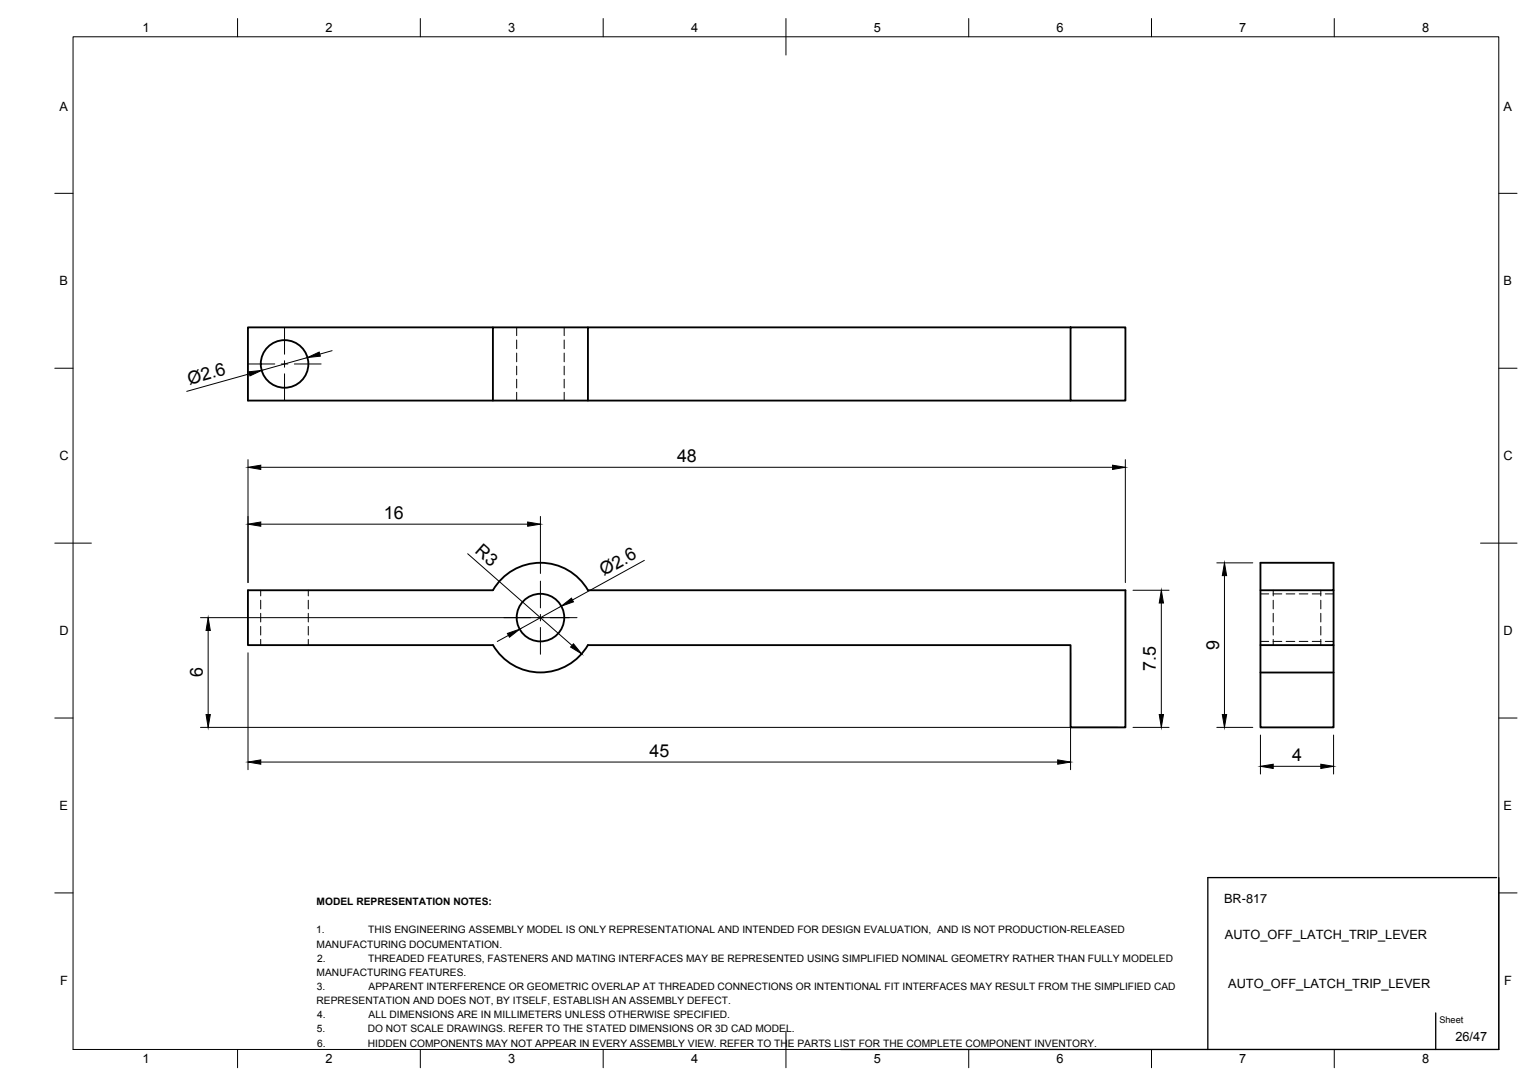
ISO-10303-21;
HEADER;
FILE_DESCRIPTION((''),'2;1');
FILE_NAME('AUTO_OFF_LATCH_TRIP_LEVER.step','2026-10-01T22:07:29-07:00',(''),(''),'','','');
FILE_SCHEMA (('AUTOMOTIVE_DESIGN { 1 0 10303 214 3 1 1 }'));
ENDSEC;
DATA;
#10=MECHANICAL_DESIGN_GEOMETRIC_PRESENTATION_REPRESENTATION('',(#558),#15484);
#488=SHAPE_REPRESENTATION_RELATIONSHIP('SRR','None',#15638,#523) ;
#523=ADVANCED_BREP_SHAPE_REPRESENTATION('',(#599),#15462) ;
#558=STYLED_ITEM('',(#15833),#599) ;
#599=MANIFOLD_SOLID_BREP('AUTO_OFF_LATCH_TRIP_LEVER',#8269) ;
#682=CYLINDRICAL_SURFACE('',#9012,0.13) ;
#683=CYLINDRICAL_SURFACE('',#9023,0.13) ;
#684=CYLINDRICAL_SURFACE('',#9025,0.3) ;
#685=CYLINDRICAL_SURFACE('',#9027,0.3) ;
#866=FACE_BOUND('',#2096,.T.) ;
#867=FACE_BOUND('',#2102,.T.) ;
#868=FACE_BOUND('',#2105,.T.) ;
#869=FACE_BOUND('',#2107,.T.) ;
#1007=CIRCLE('',#9013,0.13) ;
#1008=CIRCLE('',#9014,0.13) ;
#1009=CIRCLE('',#9019,0.3) ;
#1010=CIRCLE('',#9020,0.3) ;
#1011=CIRCLE('',#9021,0.13) ;
#1012=CIRCLE('',#9024,0.13) ;
#1013=CIRCLE('',#9026,0.3) ;
#1014=CIRCLE('',#9028,0.3) ;
#1535=FACE_OUTER_BOUND('',#2091,.T.) ;
#1536=FACE_OUTER_BOUND('',#2092,.T.) ;
#1537=FACE_OUTER_BOUND('',#2093,.T.) ;
#1538=FACE_OUTER_BOUND('',#2094,.T.) ;
#1539=FACE_OUTER_BOUND('',#2095,.T.) ;
#1540=FACE_OUTER_BOUND('',#2097,.T.) ;
#1541=FACE_OUTER_BOUND('',#2098,.T.) ;
#1542=FACE_OUTER_BOUND('',#2099,.T.) ;
#1543=FACE_OUTER_BOUND('',#2100,.T.) ;
#1544=FACE_OUTER_BOUND('',#2101,.T.) ;
#1545=FACE_OUTER_BOUND('',#2103,.T.) ;
#1546=FACE_OUTER_BOUND('',#2104,.T.) ;
#1547=FACE_OUTER_BOUND('',#2106,.T.) ;
#1548=FACE_OUTER_BOUND('',#2108,.T.) ;
#2091=EDGE_LOOP('',(#5943,#5944,#5945,#5946)) ;
#2092=EDGE_LOOP('',(#5947,#5948,#5949,#5950)) ;
#2093=EDGE_LOOP('',(#5951,#5952,#5953,#5954)) ;
#2094=EDGE_LOOP('',(#5955,#5956,#5957,#5958)) ;
#2095=EDGE_LOOP('',(#5959,#5960,#5961,#5962,#5963,#5964,#5965,#5966,#5967,
#5968)) ;
#2096=EDGE_LOOP('',(#5969)) ;
#2097=EDGE_LOOP('',(#5970,#5971,#5972,#5973)) ;
#2098=EDGE_LOOP('',(#5974,#5975,#5976,#5977)) ;
#2099=EDGE_LOOP('',(#5978,#5979,#5980,#5981)) ;
#2100=EDGE_LOOP('',(#5982,#5983,#5984,#5985)) ;
#2101=EDGE_LOOP('',(#5986,#5987,#5988,#5989)) ;
#2102=EDGE_LOOP('',(#5990)) ;
#2103=EDGE_LOOP('',(#5991,#5992,#5993,#5994)) ;
#2104=EDGE_LOOP('',(#5995,#5996,#5997,#5998,#5999,#6000,#6001,#6002,#6003,
#6004)) ;
#2105=EDGE_LOOP('',(#6005)) ;
#2106=EDGE_LOOP('',(#6006,#6007,#6008,#6009)) ;
#2107=EDGE_LOOP('',(#6010)) ;
#2108=EDGE_LOOP('',(#6011,#6012,#6013,#6014)) ;
#2649=LINE('',#13697,#3123) ;
#2650=LINE('',#13702,#3124) ;
#2651=LINE('',#13704,#3125) ;
#2652=LINE('',#13706,#3126) ;
#2653=LINE('',#13707,#3127) ;
#2654=LINE('',#13710,#3128) ;
#2655=LINE('',#13712,#3129) ;
#2656=LINE('',#13713,#3130) ;
#2657=LINE('',#13717,#3131) ;
#2658=LINE('',#13718,#3132) ;
#2659=LINE('',#13719,#3133) ;
#2660=LINE('',#13722,#3134) ;
#2661=LINE('',#13726,#3135) ;
#2662=LINE('',#13728,#3136) ;
#2663=LINE('',#13730,#3137) ;
#2664=LINE('',#13733,#3138) ;
#2665=LINE('',#13738,#3139) ;
#2666=LINE('',#13739,#3140) ;
#2667=LINE('',#13742,#3141) ;
#2668=LINE('',#13747,#3142) ;
#2669=LINE('',#13750,#3143) ;
#2670=LINE('',#13752,#3144) ;
#2671=LINE('',#13756,#3145) ;
#2672=LINE('',#13757,#3146) ;
#2673=LINE('',#13759,#3147) ;
#2674=LINE('',#13762,#3148) ;
#2675=LINE('',#13763,#3149) ;
#2676=LINE('',#13765,#3150) ;
#3123=VECTOR('',#10798,0.13) ;
#3124=VECTOR('',#10803,1.) ;
#3125=VECTOR('',#10804,1.) ;
#3126=VECTOR('',#10805,1.) ;
#3127=VECTOR('',#10806,1.) ;
#3128=VECTOR('',#10809,1.) ;
#3129=VECTOR('',#10810,1.) ;
#3130=VECTOR('',#10811,1.) ;
#3131=VECTOR('',#10814,1.) ;
#3132=VECTOR('',#10815,1.) ;
#3133=VECTOR('',#10816,1.) ;
#3134=VECTOR('',#10819,1.) ;
#3135=VECTOR('',#10822,1.) ;
#3136=VECTOR('',#10823,1.) ;
#3137=VECTOR('',#10824,1.) ;
#3138=VECTOR('',#10827,1.) ;
#3139=VECTOR('',#10832,1.) ;
#3140=VECTOR('',#10833,1.) ;
#3141=VECTOR('',#10836,0.13) ;
#3142=VECTOR('',#10843,1.) ;
#3143=VECTOR('',#10846,1.) ;
#3144=VECTOR('',#10847,1.) ;
#3145=VECTOR('',#10852,1.) ;
#3146=VECTOR('',#10853,1.) ;
#3147=VECTOR('',#10856,1.) ;
#3148=VECTOR('',#10859,1.) ;
#3149=VECTOR('',#10860,1.) ;
#3150=VECTOR('',#10863,1.) ;
#3613=VERTEX_POINT('',#13694) ;
#3614=VERTEX_POINT('',#13696) ;
#3615=VERTEX_POINT('',#13700) ;
#3616=VERTEX_POINT('',#13701) ;
#3617=VERTEX_POINT('',#13703) ;
#3618=VERTEX_POINT('',#13705) ;
#3619=VERTEX_POINT('',#13709) ;
#3620=VERTEX_POINT('',#13711) ;
#3621=VERTEX_POINT('',#13715) ;
#3622=VERTEX_POINT('',#13716) ;
#3623=VERTEX_POINT('',#13721) ;
#3624=VERTEX_POINT('',#13723) ;
#3625=VERTEX_POINT('',#13725) ;
#3626=VERTEX_POINT('',#13727) ;
#3627=VERTEX_POINT('',#13729) ;
#3628=VERTEX_POINT('',#13731) ;
#3629=VERTEX_POINT('',#13734) ;
#3630=VERTEX_POINT('',#13737) ;
#3631=VERTEX_POINT('',#13741) ;
#3632=VERTEX_POINT('',#13745) ;
#3633=VERTEX_POINT('',#13749) ;
#3634=VERTEX_POINT('',#13751) ;
#3635=VERTEX_POINT('',#13755) ;
#3636=VERTEX_POINT('',#13761) ;
#4476=EDGE_CURVE('',#3613,#3613,#1007,.T.) ;
#4477=EDGE_CURVE('',#3613,#3614,#2649,.T.) ;
#4478=EDGE_CURVE('',#3614,#3614,#1008,.T.) ;
#4479=EDGE_CURVE('',#3615,#3616,#2650,.T.) ;
#4480=EDGE_CURVE('',#3616,#3617,#2651,.T.) ;
#4481=EDGE_CURVE('',#3617,#3618,#2652,.T.) ;
#4482=EDGE_CURVE('',#3618,#3615,#2653,.T.) ;
#4483=EDGE_CURVE('',#3619,#3618,#2654,.T.) ;
#4484=EDGE_CURVE('',#3620,#3617,#2655,.T.) ;
#4485=EDGE_CURVE('',#3619,#3620,#2656,.T.) ;
#4486=EDGE_CURVE('',#3621,#3622,#2657,.T.) ;
#4487=EDGE_CURVE('',#3621,#3616,#2658,.T.) ;
#4488=EDGE_CURVE('',#3622,#3615,#2659,.T.) ;
#4489=EDGE_CURVE('',#3623,#3621,#2660,.T.) ;
#4490=EDGE_CURVE('',#3623,#3624,#1009,.T.) ;
#4491=EDGE_CURVE('',#3625,#3624,#2661,.T.) ;
#4492=EDGE_CURVE('',#3626,#3625,#2662,.T.) ;
#4493=EDGE_CURVE('',#3627,#3626,#2663,.T.) ;
#4494=EDGE_CURVE('',#3627,#3628,#1010,.T.) ;
#4495=EDGE_CURVE('',#3620,#3628,#2664,.T.) ;
#4496=EDGE_CURVE('',#3629,#3629,#1011,.T.) ;
#4497=EDGE_CURVE('',#3622,#3630,#2665,.T.) ;
#4498=EDGE_CURVE('',#3630,#3623,#2666,.T.) ;
#4499=EDGE_CURVE('',#3629,#3631,#2667,.T.) ;
#4500=EDGE_CURVE('',#3631,#3631,#1012,.T.) ;
#4501=EDGE_CURVE('',#3632,#3630,#1013,.T.) ;
#4502=EDGE_CURVE('',#3624,#3632,#2668,.T.) ;
#4503=EDGE_CURVE('',#3628,#3633,#2669,.T.) ;
#4504=EDGE_CURVE('',#3634,#3627,#2670,.T.) ;
#4505=EDGE_CURVE('',#3633,#3634,#1014,.T.) ;
#4506=EDGE_CURVE('',#3626,#3635,#2671,.T.) ;
#4507=EDGE_CURVE('',#3635,#3634,#2672,.T.) ;
#4508=EDGE_CURVE('',#3633,#3619,#2673,.T.) ;
#4509=EDGE_CURVE('',#3635,#3636,#2674,.T.) ;
#4510=EDGE_CURVE('',#3632,#3636,#2675,.T.) ;
#4511=EDGE_CURVE('',#3636,#3625,#2676,.T.) ;
#5943=ORIENTED_EDGE('',*,*,#4476,.F.) ;
#5944=ORIENTED_EDGE('',*,*,#4477,.T.) ;
#5945=ORIENTED_EDGE('',*,*,#4478,.F.) ;
#5946=ORIENTED_EDGE('',*,*,#4477,.F.) ;
#5947=ORIENTED_EDGE('',*,*,#4479,.T.) ;
#5948=ORIENTED_EDGE('',*,*,#4480,.T.) ;
#5949=ORIENTED_EDGE('',*,*,#4481,.T.) ;
#5950=ORIENTED_EDGE('',*,*,#4482,.T.) ;
#5951=ORIENTED_EDGE('',*,*,#4483,.T.) ;
#5952=ORIENTED_EDGE('',*,*,#4481,.F.) ;
#5953=ORIENTED_EDGE('',*,*,#4484,.F.) ;
#5954=ORIENTED_EDGE('',*,*,#4485,.F.) ;
#5955=ORIENTED_EDGE('',*,*,#4486,.F.) ;
#5956=ORIENTED_EDGE('',*,*,#4487,.T.) ;
#5957=ORIENTED_EDGE('',*,*,#4479,.F.) ;
#5958=ORIENTED_EDGE('',*,*,#4488,.F.) ;
#5959=ORIENTED_EDGE('',*,*,#4489,.F.) ;
#5960=ORIENTED_EDGE('',*,*,#4490,.T.) ;
#5961=ORIENTED_EDGE('',*,*,#4491,.F.) ;
#5962=ORIENTED_EDGE('',*,*,#4492,.F.) ;
#5963=ORIENTED_EDGE('',*,*,#4493,.F.) ;
#5964=ORIENTED_EDGE('',*,*,#4494,.T.) ;
#5965=ORIENTED_EDGE('',*,*,#4495,.F.) ;
#5966=ORIENTED_EDGE('',*,*,#4484,.T.) ;
#5967=ORIENTED_EDGE('',*,*,#4480,.F.) ;
#5968=ORIENTED_EDGE('',*,*,#4487,.F.) ;
#5969=ORIENTED_EDGE('',*,*,#4496,.T.) ;
#5970=ORIENTED_EDGE('',*,*,#4486,.T.) ;
#5971=ORIENTED_EDGE('',*,*,#4497,.T.) ;
#5972=ORIENTED_EDGE('',*,*,#4498,.T.) ;
#5973=ORIENTED_EDGE('',*,*,#4489,.T.) ;
#5974=ORIENTED_EDGE('',*,*,#4496,.F.) ;
#5975=ORIENTED_EDGE('',*,*,#4499,.T.) ;
#5976=ORIENTED_EDGE('',*,*,#4500,.F.) ;
#5977=ORIENTED_EDGE('',*,*,#4499,.F.) ;
#5978=ORIENTED_EDGE('',*,*,#4498,.F.) ;
#5979=ORIENTED_EDGE('',*,*,#4501,.F.) ;
#5980=ORIENTED_EDGE('',*,*,#4502,.F.) ;
#5981=ORIENTED_EDGE('',*,*,#4490,.F.) ;
#5982=ORIENTED_EDGE('',*,*,#4503,.F.) ;
#5983=ORIENTED_EDGE('',*,*,#4494,.F.) ;
#5984=ORIENTED_EDGE('',*,*,#4504,.F.) ;
#5985=ORIENTED_EDGE('',*,*,#4505,.F.) ;
#5986=ORIENTED_EDGE('',*,*,#4504,.T.) ;
#5987=ORIENTED_EDGE('',*,*,#4493,.T.) ;
#5988=ORIENTED_EDGE('',*,*,#4506,.T.) ;
#5989=ORIENTED_EDGE('',*,*,#4507,.T.) ;
#5990=ORIENTED_EDGE('',*,*,#4478,.T.) ;
#5991=ORIENTED_EDGE('',*,*,#4495,.T.) ;
#5992=ORIENTED_EDGE('',*,*,#4503,.T.) ;
#5993=ORIENTED_EDGE('',*,*,#4508,.T.) ;
#5994=ORIENTED_EDGE('',*,*,#4485,.T.) ;
#5995=ORIENTED_EDGE('',*,*,#4508,.F.) ;
#5996=ORIENTED_EDGE('',*,*,#4505,.T.) ;
#5997=ORIENTED_EDGE('',*,*,#4507,.F.) ;
#5998=ORIENTED_EDGE('',*,*,#4509,.T.) ;
#5999=ORIENTED_EDGE('',*,*,#4510,.F.) ;
#6000=ORIENTED_EDGE('',*,*,#4501,.T.) ;
#6001=ORIENTED_EDGE('',*,*,#4497,.F.) ;
#6002=ORIENTED_EDGE('',*,*,#4488,.T.) ;
#6003=ORIENTED_EDGE('',*,*,#4482,.F.) ;
#6004=ORIENTED_EDGE('',*,*,#4483,.F.) ;
#6005=ORIENTED_EDGE('',*,*,#4500,.T.) ;
#6006=ORIENTED_EDGE('',*,*,#4502,.T.) ;
#6007=ORIENTED_EDGE('',*,*,#4510,.T.) ;
#6008=ORIENTED_EDGE('',*,*,#4511,.T.) ;
#6009=ORIENTED_EDGE('',*,*,#4491,.T.) ;
#6010=ORIENTED_EDGE('',*,*,#4476,.T.) ;
#6011=ORIENTED_EDGE('',*,*,#4492,.T.) ;
#6012=ORIENTED_EDGE('',*,*,#4511,.F.) ;
#6013=ORIENTED_EDGE('',*,*,#4509,.F.) ;
#6014=ORIENTED_EDGE('',*,*,#4506,.F.) ;
#7645=PLANE('',#9015) ;
#7646=PLANE('',#9016) ;
#7647=PLANE('',#9017) ;
#7648=PLANE('',#9018) ;
#7649=PLANE('',#9022) ;
#7650=PLANE('',#9029) ;
#7651=PLANE('',#9030) ;
#7652=PLANE('',#9031) ;
#7653=PLANE('',#9032) ;
#7654=PLANE('',#9033) ;
#7922=ADVANCED_FACE('',(#1535),#682,.F.) ;
#7923=ADVANCED_FACE('',(#1536),#7645,.F.) ;
#7924=ADVANCED_FACE('',(#1537),#7646,.F.) ;
#7925=ADVANCED_FACE('',(#1538),#7647,.F.) ;
#7926=ADVANCED_FACE('',(#1539,#866),#7648,.F.) ;
#7927=ADVANCED_FACE('',(#1540),#7649,.F.) ;
#7928=ADVANCED_FACE('',(#1541),#683,.F.) ;
#7929=ADVANCED_FACE('',(#1542),#684,.T.) ;
#7930=ADVANCED_FACE('',(#1543),#685,.T.) ;
#7931=ADVANCED_FACE('',(#1544,#867),#7650,.T.) ;
#7932=ADVANCED_FACE('',(#1545),#7651,.T.) ;
#7933=ADVANCED_FACE('',(#1546,#868),#7652,.F.) ;
#7934=ADVANCED_FACE('',(#1547,#869),#7653,.F.) ;
#7935=ADVANCED_FACE('',(#1548),#7654,.F.) ;
#8269=CLOSED_SHELL('',(#7922,#7923,#7924,#7925,#7926,#7927,#7928,#7929,
#7930,#7931,#7932,#7933,#7934,#7935)) ;
#9011=AXIS2_PLACEMENT_3D('',#13692,#10792,#10793) ;
#9012=AXIS2_PLACEMENT_3D('',#13693,#10794,#10795) ;
#9013=AXIS2_PLACEMENT_3D('',#13695,#10796,#10797) ;
#9014=AXIS2_PLACEMENT_3D('',#13698,#10799,#10800) ;
#9015=AXIS2_PLACEMENT_3D('',#13699,#10801,#10802) ;
#9016=AXIS2_PLACEMENT_3D('',#13708,#10807,#10808) ;
#9017=AXIS2_PLACEMENT_3D('',#13714,#10812,#10813) ;
#9018=AXIS2_PLACEMENT_3D('',#13720,#10817,#10818) ;
#9019=AXIS2_PLACEMENT_3D('',#13724,#10820,#10821) ;
#9020=AXIS2_PLACEMENT_3D('',#13732,#10825,#10826) ;
#9021=AXIS2_PLACEMENT_3D('',#13735,#10828,#10829) ;
#9022=AXIS2_PLACEMENT_3D('',#13736,#10830,#10831) ;
#9023=AXIS2_PLACEMENT_3D('',#13740,#10834,#10835) ;
#9024=AXIS2_PLACEMENT_3D('',#13743,#10837,#10838) ;
#9025=AXIS2_PLACEMENT_3D('',#13744,#10839,#10840) ;
#9026=AXIS2_PLACEMENT_3D('',#13746,#10841,#10842) ;
#9027=AXIS2_PLACEMENT_3D('',#13748,#10844,#10845) ;
#9028=AXIS2_PLACEMENT_3D('',#13753,#10848,#10849) ;
#9029=AXIS2_PLACEMENT_3D('',#13754,#10850,#10851) ;
#9030=AXIS2_PLACEMENT_3D('',#13758,#10854,#10855) ;
#9031=AXIS2_PLACEMENT_3D('',#13760,#10857,#10858) ;
#9032=AXIS2_PLACEMENT_3D('',#13764,#10861,#10862) ;
#9033=AXIS2_PLACEMENT_3D('',#13766,#10864,#10865) ;
#10792=DIRECTION('axis',(0.,0.,1.)) ;
#10793=DIRECTION('refdir',(1.,0.,0.)) ;
#10794=DIRECTION('center_axis',(0.,0.,1.)) ;
#10795=DIRECTION('ref_axis',(1.,0.,0.)) ;
#10796=DIRECTION('center_axis',(0.,0.,1.)) ;
#10797=DIRECTION('ref_axis',(1.,0.,0.)) ;
#10798=DIRECTION('',(0.,0.,1.)) ;
#10799=DIRECTION('center_axis',(0.,0.,-1.)) ;
#10800=DIRECTION('ref_axis',(1.,0.,0.)) ;
#10801=DIRECTION('center_axis',(0.,0.,1.)) ;
#10802=DIRECTION('ref_axis',(1.,0.,0.)) ;
#10803=DIRECTION('',(0.,-1.,0.)) ;
#10804=DIRECTION('',(-1.,0.,0.)) ;
#10805=DIRECTION('',(0.,1.,0.)) ;
#10806=DIRECTION('',(1.,0.,0.)) ;
#10807=DIRECTION('center_axis',(1.,0.,0.)) ;
#10808=DIRECTION('ref_axis',(0.,0.,-1.)) ;
#10809=DIRECTION('',(0.,0.,-1.)) ;
#10810=DIRECTION('',(0.,0.,-1.)) ;
#10811=DIRECTION('',(0.,-1.,0.)) ;
#10812=DIRECTION('center_axis',(-1.,0.,0.)) ;
#10813=DIRECTION('ref_axis',(0.,0.,1.)) ;
#10814=DIRECTION('',(0.,1.,0.)) ;
#10815=DIRECTION('',(0.,0.,-1.)) ;
#10816=DIRECTION('',(0.,0.,-1.)) ;
#10817=DIRECTION('center_axis',(0.,1.,0.)) ;
#10818=DIRECTION('ref_axis',(0.,0.,1.)) ;
#10819=DIRECTION('',(-1.,0.,0.)) ;
#10820=DIRECTION('center_axis',(0.,-1.,0.)) ;
#10821=DIRECTION('ref_axis',(1.,0.,0.)) ;
#10822=DIRECTION('',(-1.,0.,0.)) ;
#10823=DIRECTION('',(0.,0.,-1.)) ;
#10824=DIRECTION('',(1.,0.,0.)) ;
#10825=DIRECTION('center_axis',(0.,-1.,0.)) ;
#10826=DIRECTION('ref_axis',(1.,0.,0.)) ;
#10827=DIRECTION('',(1.,0.,0.)) ;
#10828=DIRECTION('center_axis',(0.,1.,0.)) ;
#10829=DIRECTION('ref_axis',(1.,0.,0.)) ;
#10830=DIRECTION('center_axis',(0.,0.,1.)) ;
#10831=DIRECTION('ref_axis',(1.,0.,0.)) ;
#10832=DIRECTION('',(1.,0.,0.)) ;
#10833=DIRECTION('',(0.,-1.,0.)) ;
#10834=DIRECTION('center_axis',(0.,1.,0.)) ;
#10835=DIRECTION('ref_axis',(1.,0.,0.)) ;
#10836=DIRECTION('',(0.,1.,0.)) ;
#10837=DIRECTION('center_axis',(0.,-1.,0.)) ;
#10838=DIRECTION('ref_axis',(1.,0.,0.)) ;
#10839=DIRECTION('center_axis',(0.,1.,0.)) ;
#10840=DIRECTION('ref_axis',(1.,0.,0.)) ;
#10841=DIRECTION('center_axis',(0.,1.,0.)) ;
#10842=DIRECTION('ref_axis',(1.,0.,0.)) ;
#10843=DIRECTION('',(0.,1.,0.)) ;
#10844=DIRECTION('center_axis',(0.,1.,0.)) ;
#10845=DIRECTION('ref_axis',(1.,0.,0.)) ;
#10846=DIRECTION('',(0.,1.,0.)) ;
#10847=DIRECTION('',(0.,-1.,0.)) ;
#10848=DIRECTION('center_axis',(0.,1.,0.)) ;
#10849=DIRECTION('ref_axis',(1.,0.,0.)) ;
#10850=DIRECTION('center_axis',(0.,0.,1.)) ;
#10851=DIRECTION('ref_axis',(1.,0.,0.)) ;
#10852=DIRECTION('',(0.,1.,0.)) ;
#10853=DIRECTION('',(-1.,0.,0.)) ;
#10854=DIRECTION('center_axis',(0.,0.,1.)) ;
#10855=DIRECTION('ref_axis',(1.,0.,0.)) ;
#10856=DIRECTION('',(-1.,0.,0.)) ;
#10857=DIRECTION('center_axis',(0.,-1.,0.)) ;
#10858=DIRECTION('ref_axis',(0.,0.,-1.)) ;
#10859=DIRECTION('',(0.,0.,-1.)) ;
#10860=DIRECTION('',(1.,0.,0.)) ;
#10861=DIRECTION('center_axis',(0.,0.,1.)) ;
#10862=DIRECTION('ref_axis',(1.,0.,0.)) ;
#10863=DIRECTION('',(0.,-1.,0.)) ;
#10864=DIRECTION('center_axis',(-1.,0.,0.)) ;
#10865=DIRECTION('ref_axis',(0.,0.,1.)) ;
#13692=CARTESIAN_POINT('',(0.,0.,0.)) ;
#13693=CARTESIAN_POINT('Origin',(2.,0.7,2.3)) ;
#13694=CARTESIAN_POINT('',(1.87,0.7,2.15)) ;
#13695=CARTESIAN_POINT('Origin',(2.,0.7,2.15)) ;
#13696=CARTESIAN_POINT('',(1.87,0.7,2.45)) ;
#13697=CARTESIAN_POINT('',(1.87,0.7,2.3)) ;
#13698=CARTESIAN_POINT('Origin',(2.,0.7,2.45)) ;
#13699=CARTESIAN_POINT('Origin',(-2.45,0.7,1.7)) ;
#13700=CARTESIAN_POINT('',(-2.3,0.9,1.7)) ;
#13701=CARTESIAN_POINT('',(-2.3,0.5,1.7)) ;
#13702=CARTESIAN_POINT('',(-2.3,0.7,1.7)) ;
#13703=CARTESIAN_POINT('',(-2.6,0.5,1.7)) ;
#13704=CARTESIAN_POINT('',(-2.45,0.5,1.7)) ;
#13705=CARTESIAN_POINT('',(-2.6,0.9,1.7)) ;
#13706=CARTESIAN_POINT('',(-2.6,0.7,1.7)) ;
#13707=CARTESIAN_POINT('',(-2.45,0.9,1.7)) ;
#13708=CARTESIAN_POINT('Origin',(-2.6,0.7,2.075)) ;
#13709=CARTESIAN_POINT('',(-2.6,0.9,2.45)) ;
#13710=CARTESIAN_POINT('',(-2.6,0.9,2.075)) ;
#13711=CARTESIAN_POINT('',(-2.6,0.5,2.45)) ;
#13712=CARTESIAN_POINT('',(-2.6,0.5,2.075)) ;
#13713=CARTESIAN_POINT('',(-2.6,0.7,2.45)) ;
#13714=CARTESIAN_POINT('Origin',(-2.3,0.7,2.075)) ;
#13715=CARTESIAN_POINT('',(-2.3,0.5,2.15)) ;
#13716=CARTESIAN_POINT('',(-2.3,0.9,2.15)) ;
#13717=CARTESIAN_POINT('',(-2.3,0.7,2.15)) ;
#13718=CARTESIAN_POINT('',(-2.3,0.5,2.075)) ;
#13719=CARTESIAN_POINT('',(-2.3,0.9,2.075)) ;
#13720=CARTESIAN_POINT('Origin',(-0.1,0.5,2.3)) ;
#13721=CARTESIAN_POINT('',(0.340192378864668,0.5,2.15)) ;
#13722=CARTESIAN_POINT('',(-0.1,0.5,2.15)) ;
#13723=CARTESIAN_POINT('',(0.859807621135332,0.5,2.15)) ;
#13724=CARTESIAN_POINT('Origin',(0.6,0.5,2.3)) ;
#13725=CARTESIAN_POINT('',(2.2,0.5,2.15)) ;
#13726=CARTESIAN_POINT('',(-0.1,0.5,2.15)) ;
#13727=CARTESIAN_POINT('',(2.2,0.5,2.45)) ;
#13728=CARTESIAN_POINT('',(2.2,0.5,2.3)) ;
#13729=CARTESIAN_POINT('',(0.859807621135332,0.5,2.45)) ;
#13730=CARTESIAN_POINT('',(-0.1,0.5,2.45)) ;
#13731=CARTESIAN_POINT('',(0.340192378864668,0.5,2.45)) ;
#13732=CARTESIAN_POINT('Origin',(0.6,0.5,2.3)) ;
#13733=CARTESIAN_POINT('',(-0.1,0.5,2.45)) ;
#13734=CARTESIAN_POINT('',(0.47,0.5,2.3)) ;
#13735=CARTESIAN_POINT('Origin',(0.6,0.5,2.3)) ;
#13736=CARTESIAN_POINT('Origin',(-0.1,0.7,2.15)) ;
#13737=CARTESIAN_POINT('',(0.340192378864668,0.9,2.15)) ;
#13738=CARTESIAN_POINT('',(-0.1,0.9,2.15)) ;
#13739=CARTESIAN_POINT('',(0.340192378864668,0.7,2.15)) ;
#13740=CARTESIAN_POINT('Origin',(0.6,0.7,2.3)) ;
#13741=CARTESIAN_POINT('',(0.47,0.9,2.3)) ;
#13742=CARTESIAN_POINT('',(0.47,0.7,2.3)) ;
#13743=CARTESIAN_POINT('Origin',(0.6,0.9,2.3)) ;
#13744=CARTESIAN_POINT('Origin',(0.6,0.7,2.3)) ;
#13745=CARTESIAN_POINT('',(0.859807621135332,0.9,2.15)) ;
#13746=CARTESIAN_POINT('Origin',(0.6,0.9,2.3)) ;
#13747=CARTESIAN_POINT('',(0.859807621135332,0.7,2.15)) ;
#13748=CARTESIAN_POINT('Origin',(0.6,0.7,2.3)) ;
#13749=CARTESIAN_POINT('',(0.340192378864668,0.9,2.45)) ;
#13750=CARTESIAN_POINT('',(0.340192378864668,0.7,2.45)) ;
#13751=CARTESIAN_POINT('',(0.859807621135332,0.9,2.45)) ;
#13752=CARTESIAN_POINT('',(0.859807621135332,0.7,2.45)) ;
#13753=CARTESIAN_POINT('Origin',(0.6,0.9,2.3)) ;
#13754=CARTESIAN_POINT('Origin',(-0.1,0.7,2.45)) ;
#13755=CARTESIAN_POINT('',(2.2,0.9,2.45)) ;
#13756=CARTESIAN_POINT('',(2.2,0.7,2.45)) ;
#13757=CARTESIAN_POINT('',(-0.1,0.9,2.45)) ;
#13758=CARTESIAN_POINT('Origin',(-0.1,0.7,2.45)) ;
#13759=CARTESIAN_POINT('',(-0.1,0.9,2.45)) ;
#13760=CARTESIAN_POINT('Origin',(-0.1,0.9,2.3)) ;
#13761=CARTESIAN_POINT('',(2.2,0.9,2.15)) ;
#13762=CARTESIAN_POINT('',(2.2,0.9,2.3)) ;
#13763=CARTESIAN_POINT('',(-0.1,0.9,2.15)) ;
#13764=CARTESIAN_POINT('Origin',(-0.1,0.7,2.15)) ;
#13765=CARTESIAN_POINT('',(2.2,0.7,2.15)) ;
#13766=CARTESIAN_POINT('Origin',(2.2,0.7,2.3)) ;
#15419=UNCERTAINTY_MEASURE_WITH_UNIT(LENGTH_MEASURE(0.001),#15485,
'DISTANCE_ACCURACY_VALUE',
'Maximum model space distance between geometric entities at asserted c
onnectivities') ;
#15441=UNCERTAINTY_MEASURE_WITH_UNIT(LENGTH_MEASURE(0.001),#15485,
'DISTANCE_ACCURACY_VALUE',
'Maximum model space distance between geometric entities at asserted c
onnectivities') ;
#15462=(
GEOMETRIC_REPRESENTATION_CONTEXT(3)
GLOBAL_UNCERTAINTY_ASSIGNED_CONTEXT((#15419))
GLOBAL_UNIT_ASSIGNED_CONTEXT((#15485,#15487,#15488))
REPRESENTATION_CONTEXT('','3D')
) ;
#15484=(
GEOMETRIC_REPRESENTATION_CONTEXT(3)
GLOBAL_UNCERTAINTY_ASSIGNED_CONTEXT((#15441))
GLOBAL_UNIT_ASSIGNED_CONTEXT((#15485,#15487,#15488))
REPRESENTATION_CONTEXT('','3D')
) ;
#15485=(
LENGTH_UNIT()
NAMED_UNIT(*)
SI_UNIT(.CENTI.,.METRE.)
) ;
#15487=(
NAMED_UNIT(*)
PLANE_ANGLE_UNIT()
SI_UNIT($,.RADIAN.)
) ;
#15488=(
NAMED_UNIT(*)
SI_UNIT($,.STERADIAN.)
SOLID_ANGLE_UNIT()
) ;
#15509=SHAPE_DEFINITION_REPRESENTATION(#15566,#15638) ;
#15566=PRODUCT_DEFINITION_SHAPE('',$,#15681) ;
#15638=SHAPE_REPRESENTATION('',(#9011),#15462) ;
#15660=PRODUCT_DEFINITION_CONTEXT('part definition',#15788,'design') ;
#15681=PRODUCT_DEFINITION('AUTO_OFF_LATCH_TRIP_LEVER',
'AUTO_OFF_LATCH_TRIP_LEVER',#15723,#15660) ;
#15723=PRODUCT_DEFINITION_FORMATION('',$,#15810) ;
#15788=APPLICATION_CONTEXT(
'Core Data for Automotive Mechanical Design Process') ;
#15789=PRODUCT_CONTEXT('part definition',#15788,'mechanical') ;
#15810=PRODUCT('AUTO_OFF_LATCH_TRIP_LEVER','AUTO_OFF_LATCH_TRIP_LEVER',$,
(#15789)) ;
#15833=PRESENTATION_STYLE_ASSIGNMENT((#15845)) ;
#15845=SURFACE_STYLE_USAGE(.BOTH.,#15857) ;
#15857=SURFACE_SIDE_STYLE('',(#15869)) ;
#15869=SURFACE_STYLE_FILL_AREA(#15881) ;
#15881=FILL_AREA_STYLE('Nylon 6-6 (White)',(#15893)) ;
#15893=FILL_AREA_STYLE_COLOUR('Nylon 6-6 (White)',#15905) ;
#15905=COLOUR_RGB('Nylon 6-6 (White)', 0.31764706, 0.68627451, 0.89019608) ;
ENDSEC;
END-ISO-10303-21;
